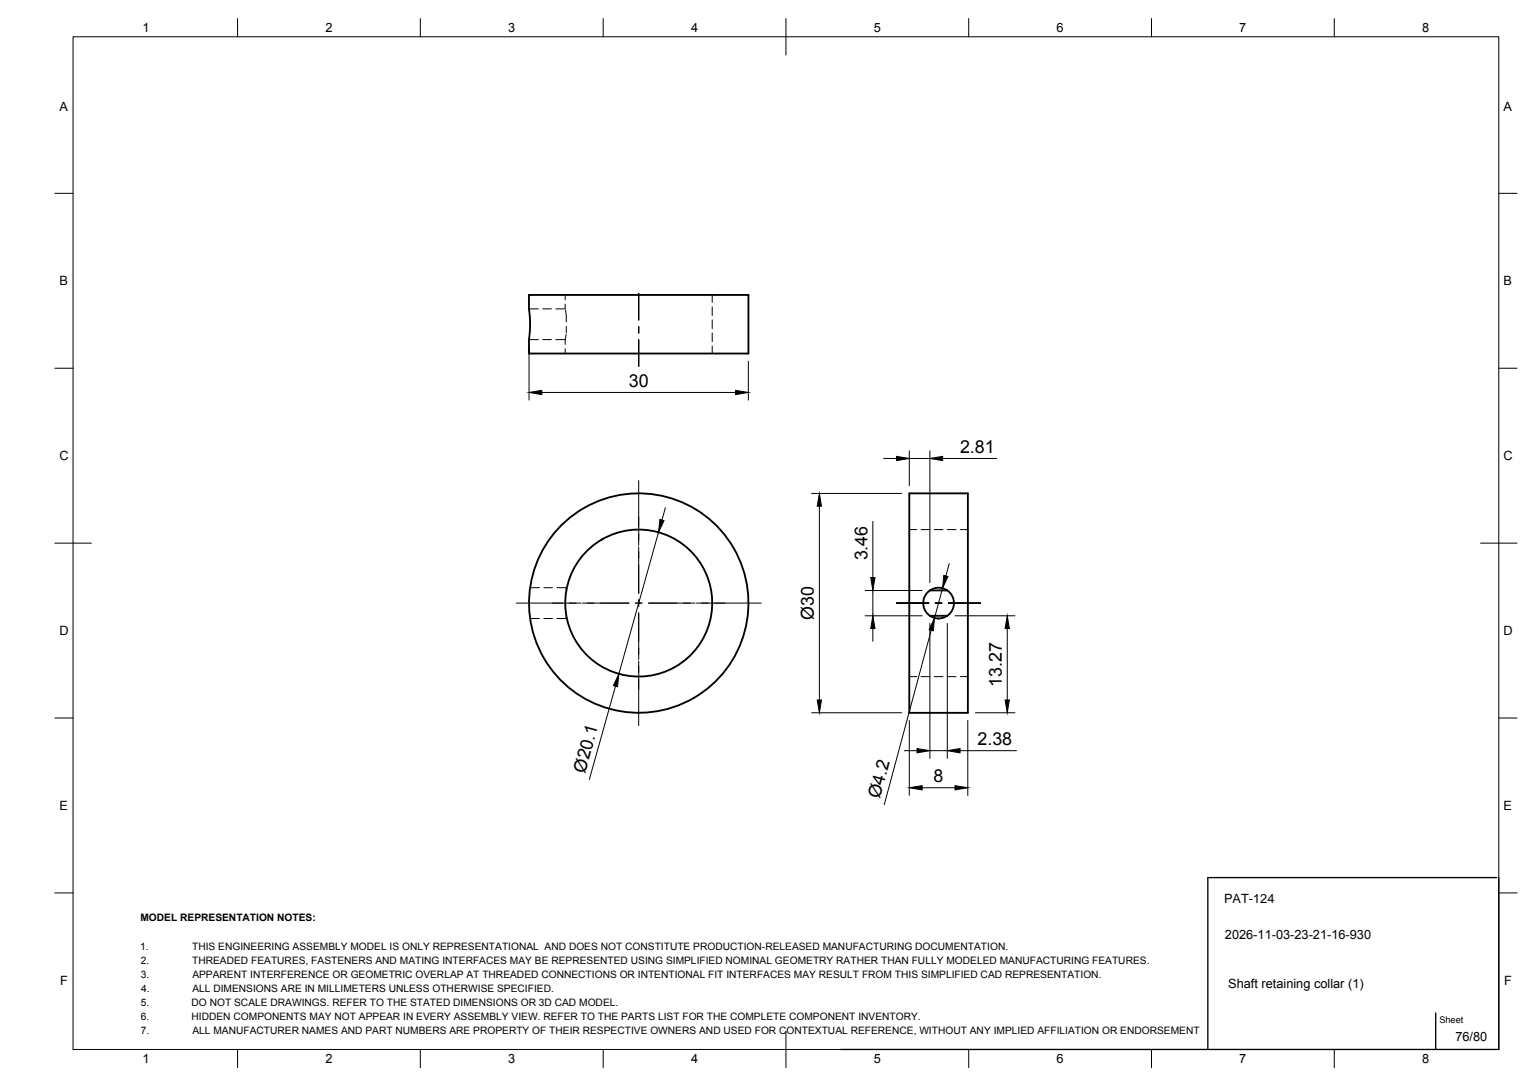
ISO-10303-21;
HEADER;
/* Generated by software containing ST-Developer
 * from STEP Tools, Inc. (www.steptools.com) 
 */

FILE_DESCRIPTION(
/* description */ ('XY cross-slide table'),
/* implementation_level */ '2;1');

FILE_NAME(
/* name */ 'Shaft retaining collar (1).step',
/* time_stamp */ '2026-10-28T03:22:46-07:00',
/* author */ (''),
/* organization */ (''),
/* preprocessor_version */ 'ST-DEVELOPER v20.2',
/* originating_system */ 'Autodesk Translation Framework v15.17.0.0',
/* authorisation */ '');

FILE_SCHEMA (('AUTOMOTIVE_DESIGN { 1 0 10303 214 3 1 1 }'));
ENDSEC;

DATA;
#10=MECHANICAL_DESIGN_GEOMETRIC_PRESENTATION_REPRESENTATION('',(#1775),#62984);
#1371=B_SPLINE_CURVE_WITH_KNOTS('',3,(#62305,#62306,#62307,#62308,#62309,
#62310,#62311,#62312),.UNSPECIFIED.,.F.,.F.,(4,2,2,4),(0.756005737987019,
0.793568827564653,0.872922520054208,0.952276212543762),.UNSPECIFIED.);
#1372=B_SPLINE_CURVE_WITH_KNOTS('',3,(#62315,#62316,#62317,#62318,#62319,
#62320,#62321,#62322,#62323,#62324,#62325,#62326,#62327,#62328),
 .UNSPECIFIED.,.F.,.F.,(4,2,2,2,2,2,4),(0.121154929624509,0.158718019202145,
0.238071711691699,0.317425404181254,0.396779096670809,0.476132789160363,
0.513695878738001),.UNSPECIFIED.);
#1373=B_SPLINE_CURVE_WITH_KNOTS('',3,(#62329,#62330,#62331,#62332,#62333,
#62334,#62335,#62336),.UNSPECIFIED.,.F.,.F.,(4,2,2,4),(0.952276212543762,
1.03162990503332,1.11098359752287,1.14854668710052),.UNSPECIFIED.);
#1374=B_SPLINE_CURVE_WITH_KNOTS('',3,(#62340,#62341,#62342,#62343,#62344,
#62345,#62346,#62347,#62348,#62349),.UNSPECIFIED.,.F.,.F.,(4,2,2,2,4),(0.,
0.0792165807733642,0.158433161546728,0.237648697074572,0.316864232602417),
 .UNSPECIFIED.);
#1375=B_SPLINE_CURVE_WITH_KNOTS('',3,(#62350,#62351,#62352,#62353,#62354,
#62355,#62356,#62357,#62358,#62359,#62360,#62361,#62362,#62363,#62364,#62365,
#62366,#62367,#62368,#62369,#62370,#62371,#62372,#62373,#62374,#62375),
 .UNSPECIFIED.,.F.,.F.,(4,2,2,2,2,2,2,2,2,2,2,2,4),(0.316864232602417,0.396079768130261,
0.475295303658105,0.554511884431469,0.633728465204833,0.712945045978197,
0.792161626751562,0.871377162279406,0.95059269780725,1.02980823333509,1.10902376886294,
1.1882403496363,1.26745693040967),.UNSPECIFIED.);
#1579=SHAPE_REPRESENTATION_RELATIONSHIP('SRR','None',#63439,#1662);
#1662=ADVANCED_BREP_SHAPE_REPRESENTATION('',(#1880),#62976);
#1775=STYLED_ITEM('',(#63912),#1880);
#1880=MANIFOLD_SOLID_BREP('Body1',#23077);
#2278=FACE_BOUND('',#5821,.T.);
#2279=FACE_BOUND('',#5823,.T.);
#2280=FACE_BOUND('',#5825,.T.);
#2281=FACE_BOUND('',#5827,.T.);
#2821=PLANE('',#26292);
#2822=PLANE('',#26296);
#2823=PLANE('',#26303);
#2824=PLANE('',#26304);
#4112=FACE_OUTER_BOUND('',#5817,.T.);
#4113=FACE_OUTER_BOUND('',#5818,.T.);
#4114=FACE_OUTER_BOUND('',#5819,.T.);
#4115=FACE_OUTER_BOUND('',#5820,.T.);
#4116=FACE_OUTER_BOUND('',#5822,.T.);
#4117=FACE_OUTER_BOUND('',#5824,.T.);
#4118=FACE_OUTER_BOUND('',#5826,.T.);
#5817=EDGE_LOOP('',(#20742,#20743));
#5818=EDGE_LOOP('',(#20744,#20745,#20746,#20747,#20748,#20749,#20750,#20751,
#20752));
#5819=EDGE_LOOP('',(#20753,#20754));
#5820=EDGE_LOOP('',(#20755,#20756,#20757,#20758));
#5821=EDGE_LOOP('',(#20759,#20760,#20761,#20762,#20763));
#5822=EDGE_LOOP('',(#20764,#20765,#20766,#20767));
#5823=EDGE_LOOP('',(#20768,#20769));
#5824=EDGE_LOOP('',(#20770));
#5825=EDGE_LOOP('',(#20771));
#5826=EDGE_LOOP('',(#20772));
#5827=EDGE_LOOP('',(#20773));
#7294=LINE('',#62300,#8781);
#7295=LINE('',#62338,#8782);
#7296=LINE('',#62377,#8783);
#7297=LINE('',#62382,#8784);
#7298=LINE('',#62388,#8785);
#8781=VECTOR('',#32435,1.);
#8782=VECTOR('',#32442,0.210000000000001);
#8783=VECTOR('',#32445,1.);
#8784=VECTOR('',#32450,1.005);
#8785=VECTOR('',#32457,1.5);
#9733=CIRCLE('',#26293,0.210000000000001);
#9734=CIRCLE('',#26295,0.210000000000001);
#9735=CIRCLE('',#26298,1.005);
#9736=CIRCLE('',#26299,1.005);
#9737=CIRCLE('',#26301,1.5);
#9738=CIRCLE('',#26302,1.5);
#11738=VERTEX_POINT('',#62298);
#11739=VERTEX_POINT('',#62299);
#11740=VERTEX_POINT('',#62303);
#11741=VERTEX_POINT('',#62304);
#11742=VERTEX_POINT('',#62313);
#11743=VERTEX_POINT('',#62337);
#11744=VERTEX_POINT('',#62339);
#11745=VERTEX_POINT('',#62379);
#11746=VERTEX_POINT('',#62381);
#11747=VERTEX_POINT('',#62385);
#11748=VERTEX_POINT('',#62387);
#14755=EDGE_CURVE('',#11738,#11739,#7294,.T.);
#14756=EDGE_CURVE('',#11738,#11739,#9733,.T.);
#14757=EDGE_CURVE('',#11740,#11741,#1371,.T.);
#14758=EDGE_CURVE('',#11742,#11740,#9734,.T.);
#14759=EDGE_CURVE('',#11739,#11742,#1372,.T.);
#14760=EDGE_CURVE('',#11741,#11738,#1373,.T.);
#14761=EDGE_CURVE('',#11741,#11743,#7295,.T.);
#14762=EDGE_CURVE('',#11744,#11743,#1374,.T.);
#14763=EDGE_CURVE('',#11743,#11744,#1375,.T.);
#14764=EDGE_CURVE('',#11742,#11740,#7296,.T.);
#14765=EDGE_CURVE('',#11745,#11745,#9735,.T.);
#14766=EDGE_CURVE('',#11745,#11746,#7297,.T.);
#14767=EDGE_CURVE('',#11746,#11746,#9736,.T.);
#14768=EDGE_CURVE('',#11747,#11747,#9737,.T.);
#14769=EDGE_CURVE('',#11747,#11748,#7298,.T.);
#14770=EDGE_CURVE('',#11748,#11748,#9738,.T.);
#20742=ORIENTED_EDGE('',*,*,#14755,.F.);
#20743=ORIENTED_EDGE('',*,*,#14756,.T.);
#20744=ORIENTED_EDGE('',*,*,#14757,.F.);
#20745=ORIENTED_EDGE('',*,*,#14758,.F.);
#20746=ORIENTED_EDGE('',*,*,#14759,.F.);
#20747=ORIENTED_EDGE('',*,*,#14756,.F.);
#20748=ORIENTED_EDGE('',*,*,#14760,.F.);
#20749=ORIENTED_EDGE('',*,*,#14761,.T.);
#20750=ORIENTED_EDGE('',*,*,#14762,.F.);
#20751=ORIENTED_EDGE('',*,*,#14763,.F.);
#20752=ORIENTED_EDGE('',*,*,#14761,.F.);
#20753=ORIENTED_EDGE('',*,*,#14764,.F.);
#20754=ORIENTED_EDGE('',*,*,#14758,.T.);
#20755=ORIENTED_EDGE('',*,*,#14765,.F.);
#20756=ORIENTED_EDGE('',*,*,#14766,.T.);
#20757=ORIENTED_EDGE('',*,*,#14767,.T.);
#20758=ORIENTED_EDGE('',*,*,#14766,.F.);
#20759=ORIENTED_EDGE('',*,*,#14759,.T.);
#20760=ORIENTED_EDGE('',*,*,#14764,.T.);
#20761=ORIENTED_EDGE('',*,*,#14757,.T.);
#20762=ORIENTED_EDGE('',*,*,#14760,.T.);
#20763=ORIENTED_EDGE('',*,*,#14755,.T.);
#20764=ORIENTED_EDGE('',*,*,#14768,.F.);
#20765=ORIENTED_EDGE('',*,*,#14769,.T.);
#20766=ORIENTED_EDGE('',*,*,#14770,.T.);
#20767=ORIENTED_EDGE('',*,*,#14769,.F.);
#20768=ORIENTED_EDGE('',*,*,#14762,.T.);
#20769=ORIENTED_EDGE('',*,*,#14763,.T.);
#20770=ORIENTED_EDGE('',*,*,#14768,.T.);
#20771=ORIENTED_EDGE('',*,*,#14765,.T.);
#20772=ORIENTED_EDGE('',*,*,#14770,.F.);
#20773=ORIENTED_EDGE('',*,*,#14767,.F.);
#21633=CYLINDRICAL_SURFACE('',#26294,0.210000000000001);
#21634=CYLINDRICAL_SURFACE('',#26297,1.005);
#21635=CYLINDRICAL_SURFACE('',#26300,1.5);
#22893=ADVANCED_FACE('',(#4112),#2821,.T.);
#22894=ADVANCED_FACE('',(#4113),#21633,.F.);
#22895=ADVANCED_FACE('',(#4114),#2822,.T.);
#22896=ADVANCED_FACE('',(#4115,#2278),#21634,.F.);
#22897=ADVANCED_FACE('',(#4116,#2279),#21635,.T.);
#22898=ADVANCED_FACE('',(#4117,#2280),#2823,.T.);
#22899=ADVANCED_FACE('',(#4118,#2281),#2824,.F.);
#23077=CLOSED_SHELL('',(#22893,#22894,#22895,#22896,#22897,#22898,#22899));
#26291=AXIS2_PLACEMENT_3D('',#62296,#32431,#32432);
#26292=AXIS2_PLACEMENT_3D('',#62297,#32433,#32434);
#26293=AXIS2_PLACEMENT_3D('',#62301,#32436,#32437);
#26294=AXIS2_PLACEMENT_3D('',#62302,#32438,#32439);
#26295=AXIS2_PLACEMENT_3D('',#62314,#32440,#32441);
#26296=AXIS2_PLACEMENT_3D('',#62376,#32443,#32444);
#26297=AXIS2_PLACEMENT_3D('',#62378,#32446,#32447);
#26298=AXIS2_PLACEMENT_3D('',#62380,#32448,#32449);
#26299=AXIS2_PLACEMENT_3D('',#62383,#32451,#32452);
#26300=AXIS2_PLACEMENT_3D('',#62384,#32453,#32454);
#26301=AXIS2_PLACEMENT_3D('',#62386,#32455,#32456);
#26302=AXIS2_PLACEMENT_3D('',#62389,#32458,#32459);
#26303=AXIS2_PLACEMENT_3D('',#62390,#32460,#32461);
#26304=AXIS2_PLACEMENT_3D('',#62391,#32462,#32463);
#32431=DIRECTION('axis',(0.,0.,1.));
#32432=DIRECTION('refdir',(1.,0.,0.));
#32433=DIRECTION('center_axis',(0.,1.,0.));
#32434=DIRECTION('ref_axis',(1.,0.,0.));
#32435=DIRECTION('',(1.,0.,0.));
#32436=DIRECTION('center_axis',(0.,1.,0.));
#32437=DIRECTION('ref_axis',(1.,0.,0.));
#32438=DIRECTION('center_axis',(0.,1.,0.));
#32439=DIRECTION('ref_axis',(1.,0.,0.));
#32440=DIRECTION('center_axis',(0.,1.,0.));
#32441=DIRECTION('ref_axis',(1.,0.,0.));
#32442=DIRECTION('',(0.,1.,0.));
#32443=DIRECTION('center_axis',(0.,1.,0.));
#32444=DIRECTION('ref_axis',(1.,0.,0.));
#32445=DIRECTION('',(-1.,0.,0.));
#32446=DIRECTION('center_axis',(1.,0.,0.));
#32447=DIRECTION('ref_axis',(0.,0.,-1.));
#32448=DIRECTION('center_axis',(-1.,0.,0.));
#32449=DIRECTION('ref_axis',(0.,0.,-1.));
#32450=DIRECTION('',(-1.,0.,0.));
#32451=DIRECTION('center_axis',(-1.,0.,0.));
#32452=DIRECTION('ref_axis',(0.,0.,-1.));
#32453=DIRECTION('center_axis',(1.,0.,0.));
#32454=DIRECTION('ref_axis',(0.,0.,-1.));
#32455=DIRECTION('center_axis',(1.,0.,0.));
#32456=DIRECTION('ref_axis',(0.,0.,-1.));
#32457=DIRECTION('',(-1.,0.,0.));
#32458=DIRECTION('center_axis',(1.,0.,0.));
#32459=DIRECTION('ref_axis',(0.,0.,-1.));
#32460=DIRECTION('center_axis',(1.,0.,0.));
#32461=DIRECTION('ref_axis',(0.,0.,-1.));
#32462=DIRECTION('center_axis',(1.,0.,0.));
#32463=DIRECTION('ref_axis',(0.,0.,-1.));
#62296=CARTESIAN_POINT('',(0.,0.,0.));
#62297=CARTESIAN_POINT('Origin',(25.8,0.99,4.));
#62298=CARTESIAN_POINT('',(25.6809411910021,0.99,4.17298843892006));
#62299=CARTESIAN_POINT('',(25.9190588089979,0.99,4.17298843892006));
#62300=CARTESIAN_POINT('',(25.4,0.99,4.17298843892006));
#62301=CARTESIAN_POINT('Origin',(25.8,0.99,4.));
#62302=CARTESIAN_POINT('Origin',(25.8,0.99,4.));
#62303=CARTESIAN_POINT('',(25.6809411910021,0.99,3.82701156107994));
#62304=CARTESIAN_POINT('',(25.59,1.005,4.));
#62305=CARTESIAN_POINT('Ctrl Pts',(25.6809411910021,0.989999999999999,3.82701156107994));
#62306=CARTESIAN_POINT('Ctrl Pts',(25.6701985776047,0.99129192197638,3.83440513468868));
#62307=CARTESIAN_POINT('Ctrl Pts',(25.6603122906273,0.992653949439047,3.84270286127439));
#62308=CARTESIAN_POINT('Ctrl Pts',(25.6329072257467,0.996748084390898,3.87010792615492));
#62309=CARTESIAN_POINT('Ctrl Pts',(25.6167579436671,0.999695893276376,3.89366983224072));
#62310=CARTESIAN_POINT('Ctrl Pts',(25.5953022060351,1.00385029472357,3.94538709536759));
#62311=CARTESIAN_POINT('Ctrl Pts',(25.59,1.005,3.97354876917015));
#62312=CARTESIAN_POINT('Ctrl Pts',(25.59,1.005,4.));
#62313=CARTESIAN_POINT('',(25.9190588089979,0.99,3.82701156107994));
#62314=CARTESIAN_POINT('Origin',(25.8,0.99,4.));
#62315=CARTESIAN_POINT('Ctrl Pts',(25.9190588089979,0.99,4.17298843892006));
#62316=CARTESIAN_POINT('Ctrl Pts',(25.9298014223953,0.991291921976381,4.16559486531132));
#62317=CARTESIAN_POINT('Ctrl Pts',(25.9396877093727,0.992653949439047,4.15729713872561));
#62318=CARTESIAN_POINT('Ctrl Pts',(25.9670927742533,0.996748084390898,4.12989207384508));
#62319=CARTESIAN_POINT('Ctrl Pts',(25.9832420563329,0.999695893276376,4.10633016775929));
#62320=CARTESIAN_POINT('Ctrl Pts',(26.0046977939649,1.00385029472357,4.05461290463241));
#62321=CARTESIAN_POINT('Ctrl Pts',(26.01,1.005,4.02645123082985));
#62322=CARTESIAN_POINT('Ctrl Pts',(26.01,1.005,3.97354876917015));
#62323=CARTESIAN_POINT('Ctrl Pts',(26.0046977939649,1.00385029472357,3.94538709536759));
#62324=CARTESIAN_POINT('Ctrl Pts',(25.9832420563329,0.999695893276376,3.89366983224072));
#62325=CARTESIAN_POINT('Ctrl Pts',(25.9670927742533,0.996748084390898,3.87010792615492));
#62326=CARTESIAN_POINT('Ctrl Pts',(25.9396877093727,0.992653949439047,3.84270286127439));
#62327=CARTESIAN_POINT('Ctrl Pts',(25.9298014223953,0.991291921976381,3.83440513468868));
#62328=CARTESIAN_POINT('Ctrl Pts',(25.9190588089979,0.99,3.82701156107994));
#62329=CARTESIAN_POINT('Ctrl Pts',(25.59,1.005,4.));
#62330=CARTESIAN_POINT('Ctrl Pts',(25.59,1.005,4.02645123082985));
#62331=CARTESIAN_POINT('Ctrl Pts',(25.5953022060351,1.00385029472357,4.05461290463241));
#62332=CARTESIAN_POINT('Ctrl Pts',(25.6167579436671,0.999695893276376,4.10633016775929));
#62333=CARTESIAN_POINT('Ctrl Pts',(25.6329072257467,0.996748084390898,4.12989207384508));
#62334=CARTESIAN_POINT('Ctrl Pts',(25.6603122906273,0.992653949439047,4.15729713872561));
#62335=CARTESIAN_POINT('Ctrl Pts',(25.6701985776047,0.991291921976381,4.16559486531132));
#62336=CARTESIAN_POINT('Ctrl Pts',(25.6809411910021,0.99,4.17298843892006));
#62337=CARTESIAN_POINT('',(25.59,1.5,4.));
#62338=CARTESIAN_POINT('',(25.59,0.99,4.));
#62339=CARTESIAN_POINT('',(25.8,1.48522725533839,4.21));
#62340=CARTESIAN_POINT('Ctrl Pts',(25.8,1.48522725533839,4.21));
#62341=CARTESIAN_POINT('Ctrl Pts',(25.7735944730755,1.48522725533839,4.21));
#62342=CARTESIAN_POINT('Ctrl Pts',(25.7454529259093,1.48600415954412,4.2047157372696));
#62343=CARTESIAN_POINT('Ctrl Pts',(25.6937237310949,1.48880073282317,4.18327376303633));
#62344=CARTESIAN_POINT('Ctrl Pts',(25.670133075872,1.49077897157582,4.16711792397039));
#62345=CARTESIAN_POINT('Ctrl Pts',(25.632882321789,1.49448481141327,4.12986716988737));
#62346=CARTESIAN_POINT('Ctrl Pts',(25.6167262899986,1.49645455657129,4.10627640830577));
#62347=CARTESIAN_POINT('Ctrl Pts',(25.5952841751738,1.49923165515646,4.0545468514059));
#62348=CARTESIAN_POINT('Ctrl Pts',(25.59,1.5,4.02640517850928));
#62349=CARTESIAN_POINT('Ctrl Pts',(25.59,1.5,4.));
#62350=CARTESIAN_POINT('Ctrl Pts',(25.59,1.5,4.));
#62351=CARTESIAN_POINT('Ctrl Pts',(25.59,1.5,3.97359482149072));
#62352=CARTESIAN_POINT('Ctrl Pts',(25.5952841751738,1.49923165515646,3.9454531485941));
#62353=CARTESIAN_POINT('Ctrl Pts',(25.6167262899986,1.49645455657129,3.89372359169423));
#62354=CARTESIAN_POINT('Ctrl Pts',(25.632882321789,1.49448481141327,3.87013283011263));
#62355=CARTESIAN_POINT('Ctrl Pts',(25.670133075872,1.49077897157582,3.83288207602961));
#62356=CARTESIAN_POINT('Ctrl Pts',(25.6937237310949,1.48880073282317,3.81672623696366));
#62357=CARTESIAN_POINT('Ctrl Pts',(25.7454529259093,1.48600415954412,3.7952842627304));
#62358=CARTESIAN_POINT('Ctrl Pts',(25.7735944730755,1.48522725533839,3.79));
#62359=CARTESIAN_POINT('Ctrl Pts',(25.8264055269245,1.48522725533839,3.79));
#62360=CARTESIAN_POINT('Ctrl Pts',(25.8545470740907,1.48600415954412,3.7952842627304));
#62361=CARTESIAN_POINT('Ctrl Pts',(25.9062762689051,1.48880073282317,3.81672623696367));
#62362=CARTESIAN_POINT('Ctrl Pts',(25.929866924128,1.49077897157582,3.83288207602961));
#62363=CARTESIAN_POINT('Ctrl Pts',(25.967117678211,1.49448481141327,3.87013283011263));
#62364=CARTESIAN_POINT('Ctrl Pts',(25.9832737100014,1.49645455657129,3.89372359169423));
#62365=CARTESIAN_POINT('Ctrl Pts',(26.0047158248262,1.49923165515646,3.9454531485941));
#62366=CARTESIAN_POINT('Ctrl Pts',(26.01,1.5,3.97359482149072));
#62367=CARTESIAN_POINT('Ctrl Pts',(26.01,1.5,4.02640517850928));
#62368=CARTESIAN_POINT('Ctrl Pts',(26.0047158248262,1.49923165515646,4.0545468514059));
#62369=CARTESIAN_POINT('Ctrl Pts',(25.9832737100014,1.49645455657129,4.10627640830577));
#62370=CARTESIAN_POINT('Ctrl Pts',(25.967117678211,1.49448481141327,4.12986716988737));
#62371=CARTESIAN_POINT('Ctrl Pts',(25.929866924128,1.49077897157582,4.16711792397039));
#62372=CARTESIAN_POINT('Ctrl Pts',(25.9062762689051,1.48880073282317,4.18327376303633));
#62373=CARTESIAN_POINT('Ctrl Pts',(25.8545470740907,1.48600415954412,4.20471573726959));
#62374=CARTESIAN_POINT('Ctrl Pts',(25.8264055269245,1.48522725533839,4.21));
#62375=CARTESIAN_POINT('Ctrl Pts',(25.8,1.48522725533839,4.21));
#62376=CARTESIAN_POINT('Origin',(25.8,0.99,4.));
#62377=CARTESIAN_POINT('',(25.4,0.99,3.82701156107994));
#62378=CARTESIAN_POINT('Origin',(25.4,0.,4.));
#62379=CARTESIAN_POINT('',(26.2,-1.23077003314309E-16,5.005));
#62380=CARTESIAN_POINT('Origin',(26.2,0.,4.));
#62381=CARTESIAN_POINT('',(25.4,-1.23077003314309E-16,5.005));
#62382=CARTESIAN_POINT('',(25.4,-1.23077003314309E-16,5.005));
#62383=CARTESIAN_POINT('Origin',(25.4,0.,4.));
#62384=CARTESIAN_POINT('Origin',(25.4,0.,4.));
#62385=CARTESIAN_POINT('',(26.2,-1.83697019872103E-16,5.5));
#62386=CARTESIAN_POINT('Origin',(26.2,0.,4.));
#62387=CARTESIAN_POINT('',(25.4,-1.83697019872103E-16,5.5));
#62388=CARTESIAN_POINT('',(25.4,-1.83697019872103E-16,5.5));
#62389=CARTESIAN_POINT('Origin',(25.4,0.,4.));
#62390=CARTESIAN_POINT('Origin',(26.2,0.,4.));
#62391=CARTESIAN_POINT('Origin',(25.4,0.,4.));
#62877=UNCERTAINTY_MEASURE_WITH_UNIT(LENGTH_MEASURE(0.001),#62985,
'DISTANCE_ACCURACY_VALUE',
'Maximum model space distance between geometric entities at asserted c
onnectivities');
#62885=UNCERTAINTY_MEASURE_WITH_UNIT(LENGTH_MEASURE(0.001),#62985,
'DISTANCE_ACCURACY_VALUE',
'Maximum model space distance between geometric entities at asserted c
onnectivities');
#62976=(
GEOMETRIC_REPRESENTATION_CONTEXT(3)
GLOBAL_UNCERTAINTY_ASSIGNED_CONTEXT((#62877))
GLOBAL_UNIT_ASSIGNED_CONTEXT((#62985,#62987,#62988))
REPRESENTATION_CONTEXT('','3D')
);
#62984=(
GEOMETRIC_REPRESENTATION_CONTEXT(3)
GLOBAL_UNCERTAINTY_ASSIGNED_CONTEXT((#62885))
GLOBAL_UNIT_ASSIGNED_CONTEXT((#62985,#62987,#62988))
REPRESENTATION_CONTEXT('','3D')
);
#62985=(
LENGTH_UNIT()
NAMED_UNIT(*)
SI_UNIT(.CENTI.,.METRE.)
);
#62987=(
NAMED_UNIT(*)
PLANE_ANGLE_UNIT()
SI_UNIT($,.RADIAN.)
);
#62988=(
NAMED_UNIT(*)
SI_UNIT($,.STERADIAN.)
SOLID_ANGLE_UNIT()
);
#63079=SHAPE_DEFINITION_REPRESENTATION(#63290,#63439);
#63290=PRODUCT_DEFINITION_SHAPE('',$,#63538);
#63439=SHAPE_REPRESENTATION('',(#26291),#62976);
#63447=PRODUCT_DEFINITION_CONTEXT('part definition',#63743,'design');
#63538=PRODUCT_DEFINITION('Shaft retaining collar (1)',
'Shaft retaining collar (1)',#63636,#63447);
#63636=PRODUCT_DEFINITION_FORMATION('',$,#63835);
#63743=APPLICATION_CONTEXT(
'Core Data for Automotive Mechanical Design Process');
#63744=PRODUCT_CONTEXT('part definition',#63743,'mechanical');
#63835=PRODUCT('Shaft retaining collar (1)','Shaft retaining collar (1)',
'Shaft retaining collar (1)',(#63744));
#63906=COLOUR_RGB('Grey',0.48,0.52,0.57);
#63907=FILL_AREA_STYLE_COLOUR('',#63906);
#63908=FILL_AREA_STYLE('',(#63907));
#63909=SURFACE_STYLE_FILL_AREA(#63908);
#63910=SURFACE_SIDE_STYLE('',(#63909));
#63911=SURFACE_STYLE_USAGE(.BOTH.,#63910);
#63912=PRESENTATION_STYLE_ASSIGNMENT((#63911));
ENDSEC;
END-ISO-10303-21;
